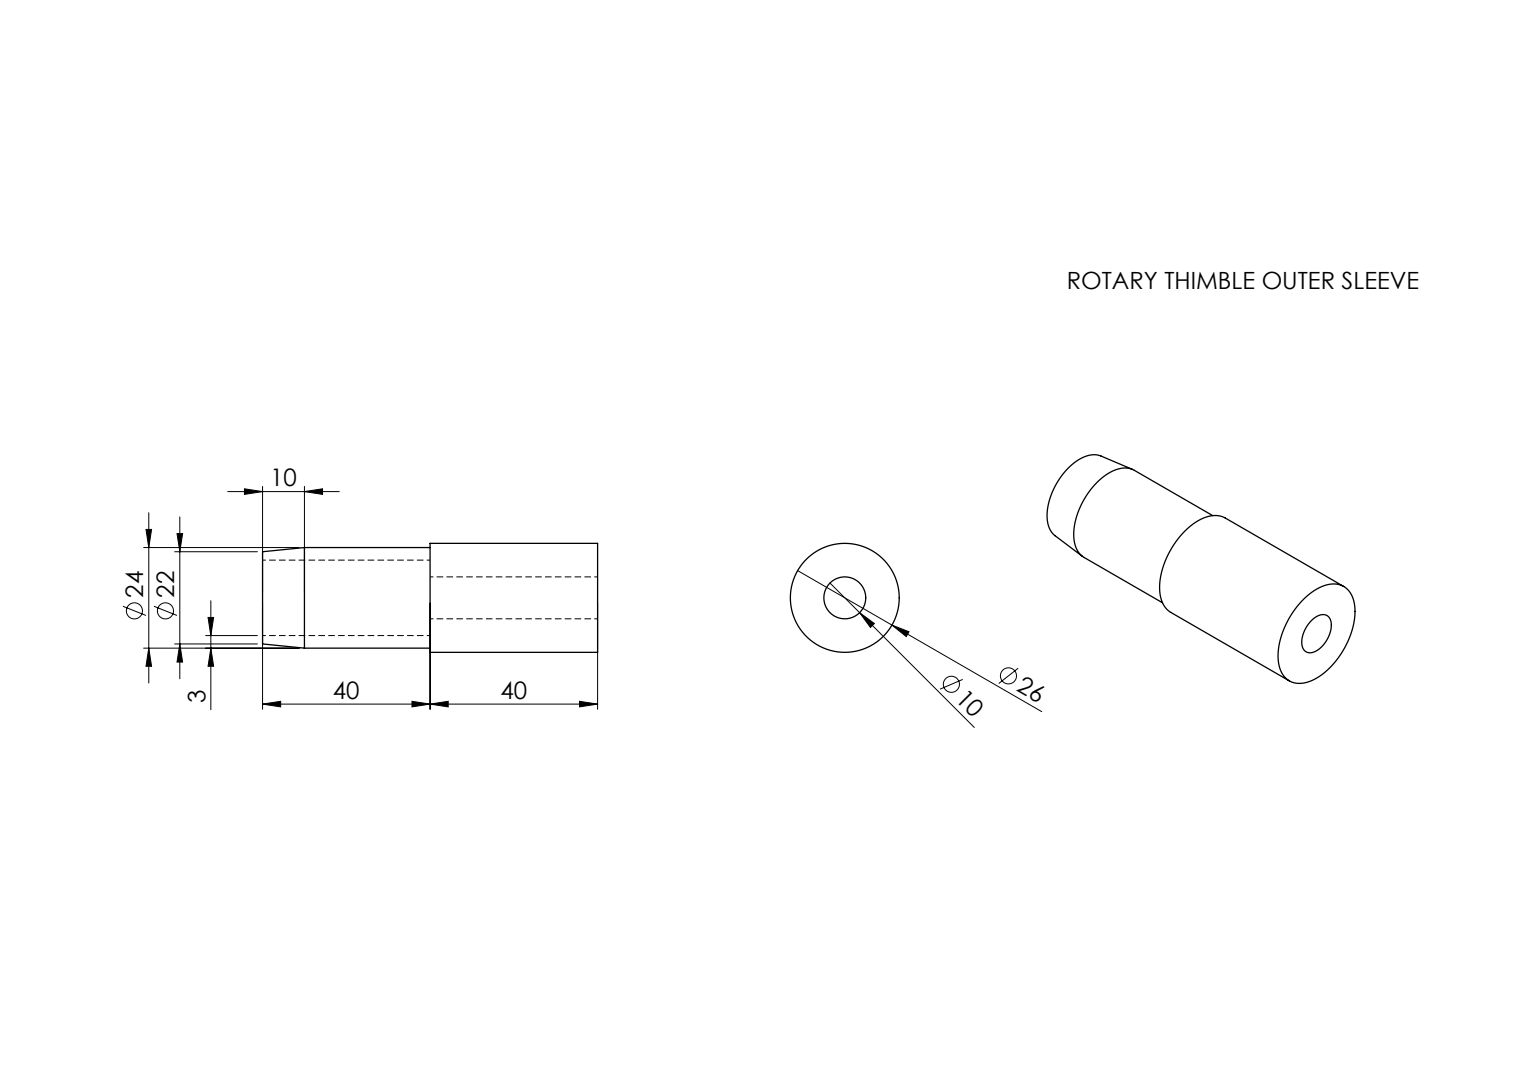
ISO-10303-21;
HEADER;
FILE_DESCRIPTION (('STEP AP214'),
    '1' );
FILE_NAME ('Rotary Thimble Outer Sleeve.step',
    '2026-10-22T12:35:56',
    ( '' ),
    ( '' ),
    'SwSTEP 2.0',
    'SolidWorks 2026',
    '' );
FILE_SCHEMA (( 'AUTOMOTIVE_DESIGN' ));
ENDSEC;

DATA;
#6=CYLINDRICAL_SURFACE ( 'NONE', #446, 5.000000000000000888 ) ;
#10=VECTOR ( 'NONE', #970, 1000.000000000000000 ) ;
#18=STYLED_ITEM ( 'NONE', ( #223 ), #2456 ) ;
#20=LINE ( 'NONE', #2499, #1316 ) ;
#22=EDGE_LOOP ( 'NONE', ( #912, #3109, #1400, #258 ) ) ;
#31=CARTESIAN_POINT ( 'NONE',  ( 100.0000000000000000, -5.826660652933936785E-15, -1.499999999999999556 ) ) ;
#37=SHAPE_REPRESENTATION_RELATIONSHIP ( 'NONE' , 'NONE' ,  #2080, #2456 ) ;
#38=EDGE_LOOP ( 'NONE', ( #1130, #2572 ) ) ;
#65=DIRECTION ( 'NONE',  ( 1.000000000000000000, 0.000000000000000000, 0.000000000000000000 ) ) ;
#83=ORIENTED_EDGE ( 'NONE', *, *, #909, .F. ) ;
#89=CARTESIAN_POINT ( 'NONE',  ( 70.00000000000032685, -6.928842772166554697E-15, 7.500000000000000000 ) ) ;
#92=CARTESIAN_POINT ( 'NONE',  ( 100.0000000000000000, -6.928842772166554697E-15, 7.500000000000000000 ) ) ;
#95=AXIS2_PLACEMENT_3D ( 'NONE', #1120, #2857, #636 ) ;
#104=EDGE_CURVE ( 'NONE', #415, #2077, #2930, .T. ) ;
#105=ORIENTED_EDGE ( 'NONE', *, *, #2070, .F. ) ;
#106=VERTEX_POINT ( 'NONE', #1616 ) ;
#108=VERTEX_POINT ( 'NONE', #3091 ) ;
#114=EDGE_LOOP ( 'NONE', ( #3092, #726, #1252, #1993 ) ) ;
#115=CIRCLE ( 'NONE', #2264, 11.00000000000000355 ) ;
#137=VERTEX_POINT ( 'NONE', #2139 ) ;
#139=DIRECTION ( 'NONE',  ( 0.000000000000000000, 0.000000000000000000, 1.000000000000000000 ) ) ;
#168=PRODUCT_CONTEXT ( 'NONE', #3176, 'mechanical' ) ;
#173=CIRCLE ( 'NONE', #1423, 12.00000000000000000 ) ;
#174=CIRCLE ( 'NONE', #2003, 12.00000000000000000 ) ;
#181=EDGE_LOOP ( 'NONE', ( #2444, #2735 ) ) ;
#183=ORIENTED_EDGE ( 'NONE', *, *, #207, .F. ) ;
#186=CARTESIAN_POINT ( 'NONE',  ( 140.0000000000000000, -6.928842772166554697E-15, 12.50000000000000000 ) ) ;
#192=EDGE_CURVE ( 'NONE', #1084, #211, #1163, .T. ) ;
#205=SURFACE_STYLE_FILL_AREA ( #2455 ) ;
#207=EDGE_CURVE ( 'NONE', #1415, #1866, #1103, .T. ) ;
#209=DIRECTION ( 'NONE',  ( 1.000000000000000000, 0.000000000000000000, 0.000000000000000000 ) ) ;
#211=VERTEX_POINT ( 'NONE', #3209 ) ;
#223=PRESENTATION_STYLE_ASSIGNMENT (( #983 ) ) ;
#230=CIRCLE ( 'NONE', #1844, 13.00000000000000178 ) ;
#236=CARTESIAN_POINT ( 'NONE',  ( 100.0000000000000000, -6.928842772166554697E-15, 19.50000000000000000 ) ) ;
#238=LINE ( 'NONE', #2000, #1057 ) ;
#240=( NAMED_UNIT ( * ) PLANE_ANGLE_UNIT ( ) SI_UNIT ( $, .RADIAN. ) );
#251=DIRECTION ( 'NONE',  ( 0.000000000000000000, 0.000000000000000000, -1.000000000000000000 ) ) ;
#255=LINE ( 'NONE', #1808, #442 ) ;
#258=ORIENTED_EDGE ( 'NONE', *, *, #2595, .F. ) ;
#271=DIRECTION ( 'NONE',  ( -1.000000000000000000, -0.000000000000000000, -0.000000000000000000 ) ) ;
#280=AXIS2_PLACEMENT_3D ( 'NONE', #2473, #2667, #2948 ) ;
#296=ADVANCED_FACE ( 'NONE', ( #1851 ), #6, .F. ) ;
#300=DIRECTION ( 'NONE',  ( 0.000000000000000000, 0.000000000000000000, -1.000000000000000000 ) ) ;
#306=DIRECTION ( 'NONE',  ( -1.000000000000000000, -0.000000000000000000, -0.000000000000000000 ) ) ;
#319=CARTESIAN_POINT ( 'NONE',  ( 100.0000000000000000, -5.826660652933936785E-15, -1.499999999999999556 ) ) ;
#322=DIRECTION ( 'NONE',  ( 0.000000000000000000, 0.000000000000000000, -1.000000000000000000 ) ) ;
#359=VERTEX_POINT ( 'NONE', #740 ) ;
#360=ADVANCED_FACE ( 'NONE', ( #1740 ), #714, .F. ) ;
#364=ORIENTED_EDGE ( 'NONE', *, *, #2262, .F. ) ;
#381=FACE_BOUND ( 'NONE', #577, .T. ) ;
#383=FACE_OUTER_BOUND ( 'NONE', #1369, .T. ) ;
#387=FACE_OUTER_BOUND ( 'NONE', #22, .T. ) ;
#402=CARTESIAN_POINT ( 'NONE',  ( 100.0000000000000000, -6.928842772166554697E-15, 20.50000000000000000 ) ) ;
#405=CYLINDRICAL_SURFACE ( 'NONE', #2026, 12.00000000000000000 ) ;
#413=CARTESIAN_POINT ( 'NONE',  ( 100.0000000000000000, -6.928842772166554697E-15, 7.500000000000000000 ) ) ;
#414=ADVANCED_FACE ( 'NONE', ( #2258 ), #2743, .F. ) ;
#415=VERTEX_POINT ( 'NONE', #482 ) ;
#421=ORIENTED_EDGE ( 'NONE', *, *, #1100, .F. ) ;
#436=EDGE_CURVE ( 'NONE', #1803, #211, #2967, .T. ) ;
#442=VECTOR ( 'NONE', #760, 1000.000000000000000 ) ;
#446=AXIS2_PLACEMENT_3D ( 'NONE', #986, #1989, #749 ) ;
#449=EDGE_LOOP ( 'NONE', ( #2891, #1302, #2981, #2325 ) ) ;
#451=ORIENTED_EDGE ( 'NONE', *, *, #3048, .T. ) ;
#457=DIRECTION ( 'NONE',  ( 0.000000000000000000, 0.000000000000000000, -1.000000000000000000 ) ) ;
#467=LINE ( 'NONE', #3149, #2202 ) ;
#482=CARTESIAN_POINT ( 'NONE',  ( 60.00000000000000000, -6.928842772166554697E-15, 16.50000000000000000 ) ) ;
#493=CIRCLE ( 'NONE', #3140, 12.00000000000000000 ) ;
#494=FACE_OUTER_BOUND ( 'NONE', #181, .T. ) ;
#495=CIRCLE ( 'NONE', #1644, 13.00000000000000178 ) ;
#501=MECHANICAL_DESIGN_GEOMETRIC_PRESENTATION_REPRESENTATION('',(#18),#1537);
#504=PLANE ( 'NONE',  #2021 ) ;
#506=( NAMED_UNIT ( * ) SI_UNIT ( $, .STERADIAN. ) SOLID_ANGLE_UNIT ( ) );
#510=EDGE_CURVE ( 'NONE', #211, #1084, #174, .T. ) ;
#528=CARTESIAN_POINT ( 'NONE',  ( 100.0000000000000000, -5.459266613189731341E-15, -4.500000000000000888 ) ) ;
#536=CYLINDRICAL_SURFACE ( 'NONE', #1581, 13.00000000000000178 ) ;
#543=CIRCLE ( 'NONE', #2666, 9.000000000000000000 ) ;
#546=VERTEX_POINT ( 'NONE', #31 ) ;
#556=CARTESIAN_POINT ( 'NONE',  ( 70.00000000000032685, -6.928842772166554697E-15, 19.50000000000000000 ) ) ;
#563=DIRECTION ( 'NONE',  ( 0.000000000000000000, 0.000000000000000000, -1.000000000000000000 ) ) ;
#570=DIRECTION ( 'NONE',  ( 1.000000000000000000, 0.000000000000000000, 0.000000000000000000 ) ) ;
#577=EDGE_LOOP ( 'NONE', ( #3165, #2114 ) ) ;
#582=DIRECTION ( 'NONE',  ( 0.9950371902099894861, 1.218569110023196515E-17, 0.09950371902099541810 ) ) ;
#590=AXIS2_PLACEMENT_3D ( 'NONE', #2153, #2814, #139 ) ;
#592=AXIS2_PLACEMENT_3D ( 'NONE', #1852, #1310, #2370 ) ;
#619=ORIENTED_EDGE ( 'NONE', *, *, #2326, .F. ) ;
#620=FACE_OUTER_BOUND ( 'NONE', #1333, .T. ) ;
#627=CARTESIAN_POINT ( 'NONE',  ( 140.0000000000000000, -6.316519372592878167E-15, 2.499999999999999556 ) ) ;
#636=DIRECTION ( 'NONE',  ( 0.000000000000000000, 0.000000000000000000, -1.000000000000000000 ) ) ;
#641=DIRECTION ( 'NONE',  ( 1.000000000000000000, 0.000000000000000000, 0.000000000000000000 ) ) ;
#665=EDGE_LOOP ( 'NONE', ( #1180, #1453, #1135, #836 ) ) ;
#692=EDGE_CURVE ( 'NONE', #3085, #1246, #230, .T. ) ;
#703=AXIS2_PLACEMENT_3D ( 'NONE', #1569, #2144, #2570 ) ;
#714=CYLINDRICAL_SURFACE ( 'NONE', #1903, 9.000000000000001776 ) ;
#715=CARTESIAN_POINT ( 'NONE',  ( 140.0000000000000000, -6.316519372592878167E-15, 2.499999999999999556 ) ) ;
#720=SURFACE_SIDE_STYLE ('',( #205 ) ) ;
#726=ORIENTED_EDGE ( 'NONE', *, *, #2442, .F. ) ;
#728=CARTESIAN_POINT ( 'NONE',  ( 100.0000000000000000, -5.459266613189731341E-15, -4.500000000000000888 ) ) ;
#740=CARTESIAN_POINT ( 'NONE',  ( 140.0000000000000000, -6.928842772166554697E-15, 20.50000000000000000 ) ) ;
#749=DIRECTION ( 'NONE',  ( 0.000000000000000000, 0.000000000000000000, 1.000000000000000000 ) ) ;
#760=DIRECTION ( 'NONE',  ( -1.000000000000000000, -0.000000000000000000, -0.000000000000000000 ) ) ;
#788=ADVANCED_FACE ( 'NONE', ( #1081 ), #2634, .T. ) ;
#793=( NAMED_UNIT ( * ) SI_UNIT ( $, .STERADIAN. ) SOLID_ANGLE_UNIT ( ) );
#806=DIRECTION ( 'NONE',  ( 1.000000000000000000, 0.000000000000000000, 0.000000000000000000 ) ) ;
#808=APPLICATION_CONTEXT ( 'automotive_design' ) ;
#811=EDGE_CURVE ( 'NONE', #546, #1226, #543, .T. ) ;
#836=ORIENTED_EDGE ( 'NONE', *, *, #2343, .F. ) ;
#849=CIRCLE ( 'NONE', #2056, 9.000000000000000000 ) ;
#860=DIRECTION ( 'NONE',  ( 1.000000000000000000, 0.000000000000000000, 0.000000000000000000 ) ) ;
#866=EDGE_CURVE ( 'NONE', #106, #137, #2406, .T. ) ;
#904=AXIS2_PLACEMENT_3D ( 'NONE', #2849, #2602, #1075 ) ;
#909=EDGE_CURVE ( 'NONE', #106, #211, #3189, .T. ) ;
#910=COLOUR_RGB ( '',0.8941176470588234615, 0.8941176470588234615, 0.8941176470588234615 ) ;
#912=ORIENTED_EDGE ( 'NONE', *, *, #2361, .F. ) ;
#944=ORIENTED_EDGE ( 'NONE', *, *, #1085, .F. ) ;
#970=DIRECTION ( 'NONE',  ( 0.9950371902099894861, 0.000000000000000000, -0.09950371902099541810 ) ) ;
#983=SURFACE_STYLE_USAGE ( .BOTH. , #720 ) ;
#986=CARTESIAN_POINT ( 'NONE',  ( 140.0000000000000000, -6.928842772166554697E-15, 7.500000000000000000 ) ) ;
#994=ADVANCED_FACE ( 'NONE', ( #1911 ), #1579, .T. ) ;
#1018=ORIENTED_EDGE ( 'NONE', *, *, #866, .F. ) ;
#1028=DIRECTION ( 'NONE',  ( 1.000000000000000000, 0.000000000000000000, 0.000000000000000000 ) ) ;
#1029=CARTESIAN_POINT ( 'NONE',  ( 140.0000000000000000, -6.928842772166554697E-15, 7.500000000000000000 ) ) ;
#1057=VECTOR ( 'NONE', #306, 1000.000000000000000 ) ;
#1064=EDGE_LOOP ( 'NONE', ( #2176, #3018 ) ) ;
#1066=DIRECTION ( 'NONE',  ( 1.000000000000000000, 0.000000000000000000, 0.000000000000000000 ) ) ;
#1075=DIRECTION ( 'NONE',  ( 0.000000000000000000, 0.000000000000000000, -1.000000000000000000 ) ) ;
#1081=FACE_OUTER_BOUND ( 'NONE', #114, .T. ) ;
#1084=VERTEX_POINT ( 'NONE', #556 ) ;
#1085=EDGE_CURVE ( 'NONE', #1226, #415, #20, .T. ) ;
#1089=DIRECTION ( 'NONE',  ( 0.000000000000000000, 0.000000000000000000, -1.000000000000000000 ) ) ;
#1100=EDGE_CURVE ( 'NONE', #2974, #2689, #1442, .T. ) ;
#1103=CIRCLE ( 'NONE', #2209, 5.000000000000000000 ) ;
#1104=EDGE_CURVE ( 'NONE', #108, #1246, #2532, .T. ) ;
#1120=CARTESIAN_POINT ( 'NONE',  ( 140.0000000000000000, -6.928842772166554697E-15, 7.500000000000000000 ) ) ;
#1121=ORIENTED_EDGE ( 'NONE', *, *, #192, .F. ) ;
#1130=ORIENTED_EDGE ( 'NONE', *, *, #104, .T. ) ;
#1131=CARTESIAN_POINT ( 'NONE',  ( 70.00000000000032685, -5.459266613189731341E-15, 19.50000000000000000 ) ) ;
#1135=ORIENTED_EDGE ( 'NONE', *, *, #1085, .T. ) ;
#1137=DIRECTION ( 'NONE',  ( 0.000000000000000000, 0.000000000000000000, -1.000000000000000000 ) ) ;
#1142=FACE_OUTER_BOUND ( 'NONE', #1994, .T. ) ;
#1163=CIRCLE ( 'NONE', #280, 12.00000000000000000 ) ;
#1167=CIRCLE ( 'NONE', #592, 9.000000000000000000 ) ;
#1173=CARTESIAN_POINT ( 'NONE',  ( 70.00000000000032685, -6.928842772166554697E-15, -4.500000000000000888 ) ) ;
#1180=ORIENTED_EDGE ( 'NONE', *, *, #1661, .F. ) ;
#1190=PRODUCT_DEFINITION_CONTEXT ( 'detailed design', #808, 'design' ) ;
#1210=CARTESIAN_POINT ( 'NONE',  ( 100.0000000000000000, -6.928842772166554697E-15, 7.500000000000000000 ) ) ;
#1224=CYLINDRICAL_SURFACE ( 'NONE', #1680, 5.000000000000000888 ) ;
#1226=VERTEX_POINT ( 'NONE', #1354 ) ;
#1242=DIRECTION ( 'NONE',  ( 0.000000000000000000, 0.000000000000000000, 1.000000000000000000 ) ) ;
#1246=VERTEX_POINT ( 'NONE', #3067 ) ;
#1252=ORIENTED_EDGE ( 'NONE', *, *, #2595, .T. ) ;
#1263=ADVANCED_FACE ( 'NONE', ( #387 ), #405, .T. ) ;
#1269=DIRECTION ( 'NONE',  ( 0.000000000000000000, 0.000000000000000000, -1.000000000000000000 ) ) ;
#1275=DIRECTION ( 'NONE',  ( 0.000000000000000000, 0.000000000000000000, -1.000000000000000000 ) ) ;
#1296=( NAMED_UNIT ( * ) PLANE_ANGLE_UNIT ( ) SI_UNIT ( $, .RADIAN. ) );
#1298=DIRECTION ( 'NONE',  ( 1.000000000000000000, 0.000000000000000000, 0.000000000000000000 ) ) ;
#1302=ORIENTED_EDGE ( 'NONE', *, *, #3048, .F. ) ;
#1306=LINE ( 'NONE', #319, #1921 ) ;
#1310=DIRECTION ( 'NONE',  ( 1.000000000000000000, 0.000000000000000000, 0.000000000000000000 ) ) ;
#1316=VECTOR ( 'NONE', #271, 1000.000000000000000 ) ;
#1317=AXIS2_PLACEMENT_3D ( 'NONE', #2581, #2862, #2829 ) ;
#1327=DIRECTION ( 'NONE',  ( -1.000000000000000000, -0.000000000000000000, -0.000000000000000000 ) ) ;
#1333=EDGE_LOOP ( 'NONE', ( #619, #1611, #2598, #83 ) ) ;
#1340=FACE_OUTER_BOUND ( 'NONE', #1064, .T. ) ;
#1354=CARTESIAN_POINT ( 'NONE',  ( 100.0000000000000000, -6.928842772166554697E-15, 16.50000000000000000 ) ) ;
#1366=DIRECTION ( 'NONE',  ( 0.000000000000000000, 0.000000000000000000, -1.000000000000000000 ) ) ;
#1369=EDGE_LOOP ( 'NONE', ( #2626, #1872, #2293, #364 ) ) ;
#1372=DIRECTION ( 'NONE',  ( 0.000000000000000000, 0.000000000000000000, -1.000000000000000000 ) ) ;
#1380=DIRECTION ( 'NONE',  ( 1.000000000000000000, 0.000000000000000000, 0.000000000000000000 ) ) ;
#1391=CARTESIAN_POINT ( 'NONE',  ( 100.0000000000000000, -6.928842772166554697E-15, 7.500000000000000000 ) ) ;
#1400=ORIENTED_EDGE ( 'NONE', *, *, #510, .T. ) ;
#1415=VERTEX_POINT ( 'NONE', #2644 ) ;
#1423=AXIS2_PLACEMENT_3D ( 'NONE', #2115, #65, #3098 ) ;
#1427=( GEOMETRIC_REPRESENTATION_CONTEXT ( 3 ) GLOBAL_UNCERTAINTY_ASSIGNED_CONTEXT ( ( #2498 ) ) GLOBAL_UNIT_ASSIGNED_CONTEXT ( ( #1452, #1664, #3164 ) ) REPRESENTATION_CONTEXT ( 'NONE', 'WORKASPACE' ) );
#1442=CIRCLE ( 'NONE', #3158, 5.000000000000000000 ) ;
#1452=( LENGTH_UNIT ( ) NAMED_UNIT ( * ) SI_UNIT ( .MILLI., .METRE. ) );
#1453=ORIENTED_EDGE ( 'NONE', *, *, #811, .T. ) ;
#1462=FILL_AREA_STYLE_COLOUR ( '', #910 ) ;
#1480=MECHANICAL_DESIGN_GEOMETRIC_PRESENTATION_REPRESENTATION('',(#2108),#1427);
#1486=PLANE ( 'NONE',  #2395 ) ;
#1496=( LENGTH_UNIT ( ) NAMED_UNIT ( * ) SI_UNIT ( .MILLI., .METRE. ) );
#1505=DIRECTION ( 'NONE',  ( -1.000000000000000000, -0.000000000000000000, -0.000000000000000000 ) ) ;
#1524=DIRECTION ( 'NONE',  ( -1.000000000000000000, -0.000000000000000000, -0.000000000000000000 ) ) ;
#1526=DIRECTION ( 'NONE',  ( 0.000000000000000000, 0.000000000000000000, -1.000000000000000000 ) ) ;
#1536=AXIS2_PLACEMENT_3D ( 'NONE', #2756, #1713, #2013 ) ;
#1537=( GEOMETRIC_REPRESENTATION_CONTEXT ( 3 ) GLOBAL_UNCERTAINTY_ASSIGNED_CONTEXT ( ( #2180 ) ) GLOBAL_UNIT_ASSIGNED_CONTEXT ( ( #1496, #1296, #793 ) ) REPRESENTATION_CONTEXT ( 'NONE', 'WORKASPACE' ) );
#1540=PRODUCT_DEFINITION_FORMATION_WITH_SPECIFIED_SOURCE ( 'ANY', '', #2617, .NOT_KNOWN. ) ;
#1565=EDGE_LOOP ( 'NONE', ( #2027, #1018, #3065, #1121 ) ) ;
#1569=CARTESIAN_POINT ( 'NONE',  ( 140.0000000000000000, -6.928842772166554697E-15, 7.500000000000000000 ) ) ;
#1579=CONICAL_SURFACE ( 'NONE', #1635, 12.00000000000000000, 0.09966865249115851311 ) ;
#1581=AXIS2_PLACEMENT_3D ( 'NONE', #2731, #1524, #1242 ) ;
#1586=VECTOR ( 'NONE', #2478, 1000.000000000000000 ) ;
#1590=ADVANCED_FACE ( 'NONE', ( #2046, #3035 ), #504, .T. ) ;
#1603=CARTESIAN_POINT ( 'NONE',  ( 100.0000000000000000, -6.928842772166554697E-15, 7.500000000000000000 ) ) ;
#1610=ORIENTED_EDGE ( 'NONE', *, *, #2361, .T. ) ;
#1611=ORIENTED_EDGE ( 'NONE', *, *, #2298, .T. ) ;
#1616=CARTESIAN_POINT ( 'NONE',  ( 60.00000000000000000, -6.928842772166554697E-15, -3.500000000000003109 ) ) ;
#1635=AXIS2_PLACEMENT_3D ( 'NONE', #1719, #2700, #457 ) ;
#1644=AXIS2_PLACEMENT_3D ( 'NONE', #1902, #860, #2091 ) ;
#1658=ORIENTED_EDGE ( 'NONE', *, *, #1100, .T. ) ;
#1661=EDGE_CURVE ( 'NONE', #546, #2077, #1306, .T. ) ;
#1664=( NAMED_UNIT ( * ) PLANE_ANGLE_UNIT ( ) SI_UNIT ( $, .RADIAN. ) );
#1680=AXIS2_PLACEMENT_3D ( 'NONE', #1962, #2753, #2271 ) ;
#1702=CIRCLE ( 'NONE', #2564, 13.00000000000000178 ) ;
#1713=DIRECTION ( 'NONE',  ( -1.000000000000000000, -0.000000000000000000, -0.000000000000000000 ) ) ;
#1718=ADVANCED_FACE ( 'NONE', ( #381, #1142 ), #1898, .F. ) ;
#1719=CARTESIAN_POINT ( 'NONE',  ( 70.00000000000032685, -6.928842772166554697E-15, 7.500000000000000000 ) ) ;
#1723=FACE_BOUND ( 'NONE', #38, .T. ) ;
#1730=CIRCLE ( 'NONE', #95, 5.000000000000000000 ) ;
#1731=DIRECTION ( 'NONE',  ( -1.000000000000000000, -0.000000000000000000, -0.000000000000000000 ) ) ;
#1736=CARTESIAN_POINT ( 'NONE',  ( 60.00000000000000000, -6.928842772166554697E-15, 7.500000000000000000 ) ) ;
#1740=FACE_OUTER_BOUND ( 'NONE', #665, .T. ) ;
#1746=AXIS2_PLACEMENT_3D ( 'NONE', #92, #2079, #2557 ) ;
#1776=ADVANCED_FACE ( 'NONE', ( #494, #1723 ), #1486, .F. ) ;
#1794=DIRECTION ( 'NONE',  ( 1.000000000000000000, 0.000000000000000000, 0.000000000000000000 ) ) ;
#1803=VERTEX_POINT ( 'NONE', #528 ) ;
#1808=CARTESIAN_POINT ( 'NONE',  ( 140.0000000000000000, -6.928842772166554697E-15, 20.50000000000000000 ) ) ;
#1810=CARTESIAN_POINT ( 'NONE',  ( 140.0000000000000000, -5.336801933274995404E-15, -5.500000000000001776 ) ) ;
#1811=ORIENTED_EDGE ( 'NONE', *, *, #2070, .T. ) ;
#1819=EDGE_LOOP ( 'NONE', ( #451, #2655 ) ) ;
#1826=ADVANCED_FACE ( 'NONE', ( #2240 ), #1224, .F. ) ;
#1837=DIRECTION ( 'NONE',  ( 1.000000000000000000, 0.000000000000000000, 0.000000000000000000 ) ) ;
#1844=AXIS2_PLACEMENT_3D ( 'NONE', #2486, #1298, #3049 ) ;
#1851=FACE_OUTER_BOUND ( 'NONE', #2388, .T. ) ;
#1852=CARTESIAN_POINT ( 'NONE',  ( 60.00000000000000000, -6.928842772166554697E-15, 7.500000000000000000 ) ) ;
#1855=EDGE_LOOP ( 'NONE', ( #2272, #1610 ) ) ;
#1866=VERTEX_POINT ( 'NONE', #2978 ) ;
#1868=DIRECTION ( 'NONE',  ( 0.000000000000000000, 0.000000000000000000, 1.000000000000000000 ) ) ;
#1872=ORIENTED_EDGE ( 'NONE', *, *, #1104, .T. ) ;
#1888=VECTOR ( 'NONE', #2166, 1000.000000000000000 ) ;
#1898=PLANE ( 'NONE',  #2748 ) ;
#1901=ORIENTED_EDGE ( 'NONE', *, *, #2191, .F. ) ;
#1902=CARTESIAN_POINT ( 'NONE',  ( 140.0000000000000000, -6.928842772166554697E-15, 7.500000000000000000 ) ) ;
#1903=AXIS2_PLACEMENT_3D ( 'NONE', #1210, #1505, #2449 ) ;
#1911=FACE_OUTER_BOUND ( 'NONE', #1565, .T. ) ;
#1921=VECTOR ( 'NONE', #2306, 1000.000000000000000 ) ;
#1959=( LENGTH_UNIT ( ) NAMED_UNIT ( * ) SI_UNIT ( .MILLI., .METRE. ) );
#1962=CARTESIAN_POINT ( 'NONE',  ( 140.0000000000000000, -6.928842772166554697E-15, 7.500000000000000000 ) ) ;
#1987=ADVANCED_FACE ( 'NONE', ( #620 ), #2141, .T. ) ;
#1989=DIRECTION ( 'NONE',  ( -1.000000000000000000, -0.000000000000000000, -0.000000000000000000 ) ) ;
#1993=ORIENTED_EDGE ( 'NONE', *, *, #192, .T. ) ;
#1994=EDGE_LOOP ( 'NONE', ( #2692, #2519 ) ) ;
#2000=CARTESIAN_POINT ( 'NONE',  ( 140.0000000000000000, -6.928842772166554697E-15, 12.50000000000000000 ) ) ;
#2003=AXIS2_PLACEMENT_3D ( 'NONE', #89, #2075, #300 ) ;
#2013=DIRECTION ( 'NONE',  ( 0.000000000000000000, 0.000000000000000000, 1.000000000000000000 ) ) ;
#2021=AXIS2_PLACEMENT_3D ( 'NONE', #1029, #806, #251 ) ;
#2026=AXIS2_PLACEMENT_3D ( 'NONE', #1391, #1327, #1868 ) ;
#2027=ORIENTED_EDGE ( 'NONE', *, *, #2298, .F. ) ;
#2046=FACE_OUTER_BOUND ( 'NONE', #1819, .T. ) ;
#2051=AXIS2_PLACEMENT_3D ( 'NONE', #2685, #1731, #2647 ) ;
#2056=AXIS2_PLACEMENT_3D ( 'NONE', #1603, #2368, #1089 ) ;
#2070=EDGE_CURVE ( 'NONE', #2689, #2974, #1730, .T. ) ;
#2075=DIRECTION ( 'NONE',  ( 1.000000000000000000, -0.000000000000000000, -0.000000000000000000 ) ) ;
#2077=VERTEX_POINT ( 'NONE', #2609 ) ;
#2079=DIRECTION ( 'NONE',  ( 1.000000000000000000, 0.000000000000000000, 0.000000000000000000 ) ) ;
#2080=SHAPE_REPRESENTATION ( 'Rotary Thimble Outer Sleeve', ( #2878 ), #2989 ) ;
#2091=DIRECTION ( 'NONE',  ( 0.000000000000000000, 0.000000000000000000, -1.000000000000000000 ) ) ;
#2095=SHAPE_DEFINITION_REPRESENTATION ( #2977, #2080 ) ;
#2108=STYLED_ITEM('',(#3243),#3178);
#2114=ORIENTED_EDGE ( 'NONE', *, *, #207, .T. ) ;
#2115=CARTESIAN_POINT ( 'NONE',  ( 100.0000000000000000, -6.928842772166554697E-15, 7.500000000000000000 ) ) ;
#2127=CYLINDRICAL_SURFACE ( 'NONE', #703, 13.00000000000000178 ) ;
#2139=CARTESIAN_POINT ( 'NONE',  ( 60.00000000000000000, -5.520498953147098126E-15, 18.50000000000000355 ) ) ;
#2141=CONICAL_SURFACE ( 'NONE', #3068, 12.00000000000000000, 0.09966865249115851311 ) ;
#2144=DIRECTION ( 'NONE',  ( -1.000000000000000000, -0.000000000000000000, -0.000000000000000000 ) ) ;
#2153=CARTESIAN_POINT ( 'NONE',  ( 100.0000000000000000, -6.928842772166554697E-15, 7.500000000000000000 ) ) ;
#2156=ORIENTED_EDGE ( 'NONE', *, *, #1661, .T. ) ;
#2166=DIRECTION ( 'NONE',  ( -1.000000000000000000, -0.000000000000000000, -0.000000000000000000 ) ) ;
#2172=ADVANCED_FACE ( 'NONE', ( #2760 ), #536, .T. ) ;
#2176=ORIENTED_EDGE ( 'NONE', *, *, #692, .F. ) ;
#2180=UNCERTAINTY_MEASURE_WITH_UNIT (LENGTH_MEASURE( 1.000000000000000082E-05 ), #1496, 'distance_accuracy_value', 'NONE');
#2191=EDGE_CURVE ( 'NONE', #1866, #1415, #3084, .T. ) ;
#2193=EDGE_CURVE ( 'NONE', #2689, #1866, #238, .T. ) ;
#2195=ORIENTED_EDGE ( 'NONE', *, *, #2193, .F. ) ;
#2202=VECTOR ( 'NONE', #3183, 1000.000000000000000 ) ;
#2204=DIRECTION ( 'NONE',  ( 0.000000000000000000, 0.000000000000000000, -1.000000000000000000 ) ) ;
#2209=AXIS2_PLACEMENT_3D ( 'NONE', #2961, #2715, #2204 ) ;
#2240=FACE_OUTER_BOUND ( 'NONE', #3148, .T. ) ;
#2258=FACE_OUTER_BOUND ( 'NONE', #2754, .T. ) ;
#2262=EDGE_CURVE ( 'NONE', #359, #3085, #255, .T. ) ;
#2263=LINE ( 'NONE', #1131, #2668 ) ;
#2264=AXIS2_PLACEMENT_3D ( 'NONE', #3080, #3112, #1372 ) ;
#2271=DIRECTION ( 'NONE',  ( 0.000000000000000000, 0.000000000000000000, 1.000000000000000000 ) ) ;
#2272=ORIENTED_EDGE ( 'NONE', *, *, #2442, .T. ) ;
#2277=DIRECTION ( 'NONE',  ( 0.000000000000000000, 0.000000000000000000, -1.000000000000000000 ) ) ;
#2291=CARTESIAN_POINT ( 'NONE',  ( 100.0000000000000000, -6.928842772166554697E-15, 7.500000000000000000 ) ) ;
#2293=ORIENTED_EDGE ( 'NONE', *, *, #2906, .T. ) ;
#2298=EDGE_CURVE ( 'NONE', #137, #1084, #2263, .T. ) ;
#2306=DIRECTION ( 'NONE',  ( -1.000000000000000000, -0.000000000000000000, -0.000000000000000000 ) ) ;
#2321=CARTESIAN_POINT ( 'NONE',  ( 100.0000000000000000, -6.928842772166554697E-15, 7.500000000000000000 ) ) ;
#2325=ORIENTED_EDGE ( 'NONE', *, *, #692, .T. ) ;
#2326=EDGE_CURVE ( 'NONE', #137, #106, #115, .T. ) ;
#2336=PLANE ( 'NONE',  #1746 ) ;
#2343=EDGE_CURVE ( 'NONE', #2077, #415, #1167, .T. ) ;
#2361=EDGE_CURVE ( 'NONE', #1803, #2769, #493, .T. ) ;
#2368=DIRECTION ( 'NONE',  ( 1.000000000000000000, 0.000000000000000000, 0.000000000000000000 ) ) ;
#2370=DIRECTION ( 'NONE',  ( 0.000000000000000000, 0.000000000000000000, -1.000000000000000000 ) ) ;
#2388=EDGE_LOOP ( 'NONE', ( #2855, #1658, #2980, #183 ) ) ;
#2392=ADVANCED_FACE ( 'NONE', ( #2869, #1340 ), #2336, .F. ) ;
#2395=AXIS2_PLACEMENT_3D ( 'NONE', #1736, #209, #1269 ) ;
#2406=CIRCLE ( 'NONE', #2051, 11.00000000000000355 ) ;
#2413=ORIENTED_EDGE ( 'NONE', *, *, #3060, .T. ) ;
#2442=EDGE_CURVE ( 'NONE', #2769, #1803, #173, .T. ) ;
#2444=ORIENTED_EDGE ( 'NONE', *, *, #866, .T. ) ;
#2449=DIRECTION ( 'NONE',  ( 0.000000000000000000, 0.000000000000000000, 1.000000000000000000 ) ) ;
#2455=FILL_AREA_STYLE ('',( #1462 ) ) ;
#2456=ADVANCED_BREP_SHAPE_REPRESENTATION ( '', ( #3178, #2878 ), #2989 ) ;
#2473=CARTESIAN_POINT ( 'NONE',  ( 70.00000000000032685, -6.928842772166554697E-15, 7.500000000000000000 ) ) ;
#2476=ORIENTED_EDGE ( 'NONE', *, *, #2714, .T. ) ;
#2478=DIRECTION ( 'NONE',  ( -1.000000000000000000, -0.000000000000000000, -0.000000000000000000 ) ) ;
#2482=CARTESIAN_POINT ( 'NONE',  ( 100.0000000000000000, -6.928842772166554697E-15, 7.500000000000000000 ) ) ;
#2486=CARTESIAN_POINT ( 'NONE',  ( 100.0000000000000000, -6.928842772166554697E-15, 7.500000000000000000 ) ) ;
#2498=UNCERTAINTY_MEASURE_WITH_UNIT (LENGTH_MEASURE( 1.000000000000000082E-05 ), #1452, 'distance_accuracy_value', 'NONE');
#2499=CARTESIAN_POINT ( 'NONE',  ( 100.0000000000000000, -6.928842772166554697E-15, 16.50000000000000000 ) ) ;
#2519=ORIENTED_EDGE ( 'NONE', *, *, #811, .F. ) ;
#2532=LINE ( 'NONE', #1810, #2844 ) ;
#2557=DIRECTION ( 'NONE',  ( 0.000000000000000000, 0.000000000000000000, -1.000000000000000000 ) ) ;
#2564=AXIS2_PLACEMENT_3D ( 'NONE', #2291, #1028, #1275 ) ;
#2570=DIRECTION ( 'NONE',  ( 0.000000000000000000, 0.000000000000000000, 1.000000000000000000 ) ) ;
#2572=ORIENTED_EDGE ( 'NONE', *, *, #2343, .T. ) ;
#2581=CARTESIAN_POINT ( 'NONE',  ( 60.00000000000000000, -6.928842772166554697E-15, 7.500000000000000000 ) ) ;
#2595=EDGE_CURVE ( 'NONE', #2769, #1084, #467, .T. ) ;
#2598=ORIENTED_EDGE ( 'NONE', *, *, #510, .F. ) ;
#2602=DIRECTION ( 'NONE',  ( 1.000000000000000000, 0.000000000000000000, 0.000000000000000000 ) ) ;
#2609=CARTESIAN_POINT ( 'NONE',  ( 60.00000000000000000, -5.826660652933936785E-15, -1.499999999999999556 ) ) ;
#2617=PRODUCT ( 'Rotary Thimble Outer Sleeve', 'Rotary Thimble Outer Sleeve', '', ( #168 ) ) ;
#2626=ORIENTED_EDGE ( 'NONE', *, *, #3019, .F. ) ;
#2634=CYLINDRICAL_SURFACE ( 'NONE', #590, 12.00000000000000000 ) ;
#2644=CARTESIAN_POINT ( 'NONE',  ( 100.0000000000000000, -6.316519372592878167E-15, 2.499999999999999556 ) ) ;
#2647=DIRECTION ( 'NONE',  ( 0.000000000000000000, 0.000000000000000000, -1.000000000000000000 ) ) ;
#2655=ORIENTED_EDGE ( 'NONE', *, *, #3019, .T. ) ;
#2658=UNCERTAINTY_MEASURE_WITH_UNIT (LENGTH_MEASURE( 1.000000000000000082E-05 ), #1959, 'distance_accuracy_value', 'NONE');
#2659=LINE ( 'NONE', #715, #1888 ) ;
#2666=AXIS2_PLACEMENT_3D ( 'NONE', #3086, #1380, #1137 ) ;
#2667=DIRECTION ( 'NONE',  ( 1.000000000000000000, -0.000000000000000000, -0.000000000000000000 ) ) ;
#2668=VECTOR ( 'NONE', #582, 1000.000000000000000 ) ;
#2685=CARTESIAN_POINT ( 'NONE',  ( 60.00000000000000000, -6.928842772166554697E-15, 7.500000000000000000 ) ) ;
#2689=VERTEX_POINT ( 'NONE', #186 ) ;
#2692=ORIENTED_EDGE ( 'NONE', *, *, #3060, .F. ) ;
#2700=DIRECTION ( 'NONE',  ( 1.000000000000000000, -0.000000000000000000, -0.000000000000000000 ) ) ;
#2714=EDGE_CURVE ( 'NONE', #2974, #1415, #2659, .T. ) ;
#2715=DIRECTION ( 'NONE',  ( 1.000000000000000000, 0.000000000000000000, 0.000000000000000000 ) ) ;
#2719=ORIENTED_EDGE ( 'NONE', *, *, #104, .F. ) ;
#2731=CARTESIAN_POINT ( 'NONE',  ( 140.0000000000000000, -6.928842772166554697E-15, 7.500000000000000000 ) ) ;
#2735=ORIENTED_EDGE ( 'NONE', *, *, #2326, .T. ) ;
#2743=CYLINDRICAL_SURFACE ( 'NONE', #1536, 9.000000000000001776 ) ;
#2748=AXIS2_PLACEMENT_3D ( 'NONE', #413, #641, #1366 ) ;
#2753=DIRECTION ( 'NONE',  ( -1.000000000000000000, -0.000000000000000000, -0.000000000000000000 ) ) ;
#2754=EDGE_LOOP ( 'NONE', ( #2413, #2156, #2719, #944 ) ) ;
#2756=CARTESIAN_POINT ( 'NONE',  ( 100.0000000000000000, -6.928842772166554697E-15, 7.500000000000000000 ) ) ;
#2760=FACE_OUTER_BOUND ( 'NONE', #449, .T. ) ;
#2769=VERTEX_POINT ( 'NONE', #236 ) ;
#2793=DIRECTION ( 'NONE',  ( -1.000000000000000000, -0.000000000000000000, -0.000000000000000000 ) ) ;
#2799=DIRECTION ( 'NONE',  ( 0.000000000000000000, 0.000000000000000000, 1.000000000000000000 ) ) ;
#2814=DIRECTION ( 'NONE',  ( -1.000000000000000000, -0.000000000000000000, -0.000000000000000000 ) ) ;
#2829=DIRECTION ( 'NONE',  ( 0.000000000000000000, 0.000000000000000000, -1.000000000000000000 ) ) ;
#2844=VECTOR ( 'NONE', #2793, 1000.000000000000000 ) ;
#2849=CARTESIAN_POINT ( 'NONE',  ( 140.0000000000000000, -6.928842772166554697E-15, 7.500000000000000000 ) ) ;
#2854=PRODUCT_DEFINITION ( 'UNKNOWN', '', #1540, #1190 ) ;
#2855=ORIENTED_EDGE ( 'NONE', *, *, #2714, .F. ) ;
#2857=DIRECTION ( 'NONE',  ( 1.000000000000000000, 0.000000000000000000, 0.000000000000000000 ) ) ;
#2862=DIRECTION ( 'NONE',  ( 1.000000000000000000, 0.000000000000000000, 0.000000000000000000 ) ) ;
#2869=FACE_BOUND ( 'NONE', #1855, .T. ) ;
#2873=CARTESIAN_POINT ( 'NONE',  ( 70.00000000000032685, -6.928842772166554697E-15, 7.500000000000000000 ) ) ;
#2878=AXIS2_PLACEMENT_3D ( 'NONE', #3071, #2799, #1837 ) ;
#2891=ORIENTED_EDGE ( 'NONE', *, *, #1104, .F. ) ;
#2906=EDGE_CURVE ( 'NONE', #1246, #3085, #1702, .T. ) ;
#2930=CIRCLE ( 'NONE', #1317, 9.000000000000000000 ) ;
#2932=AXIS2_PLACEMENT_3D ( 'NONE', #2482, #570, #2277 ) ;
#2948=DIRECTION ( 'NONE',  ( 0.000000000000000000, 0.000000000000000000, -1.000000000000000000 ) ) ;
#2959=ADVANCED_FACE ( 'NONE', ( #383 ), #2127, .T. ) ;
#2961=CARTESIAN_POINT ( 'NONE',  ( 100.0000000000000000, -6.928842772166554697E-15, 7.500000000000000000 ) ) ;
#2967=LINE ( 'NONE', #728, #1586 ) ;
#2974=VERTEX_POINT ( 'NONE', #627 ) ;
#2977=PRODUCT_DEFINITION_SHAPE ( 'NONE', 'NONE',  #2854 ) ;
#2978=CARTESIAN_POINT ( 'NONE',  ( 100.0000000000000000, -6.928842772166554697E-15, 12.50000000000000000 ) ) ;
#2980=ORIENTED_EDGE ( 'NONE', *, *, #2193, .T. ) ;
#2981=ORIENTED_EDGE ( 'NONE', *, *, #2262, .T. ) ;
#2983=CIRCLE ( 'NONE', #904, 13.00000000000000178 ) ;
#2989=( GEOMETRIC_REPRESENTATION_CONTEXT ( 3 ) GLOBAL_UNCERTAINTY_ASSIGNED_CONTEXT ( ( #2658 ) ) GLOBAL_UNIT_ASSIGNED_CONTEXT ( ( #1959, #240, #506 ) ) REPRESENTATION_CONTEXT ( 'NONE', 'WORKASPACE' ) );
#3008=EDGE_LOOP ( 'NONE', ( #105, #421 ) ) ;
#3018=ORIENTED_EDGE ( 'NONE', *, *, #2906, .F. ) ;
#3019=EDGE_CURVE ( 'NONE', #108, #359, #495, .T. ) ;
#3021=CARTESIAN_POINT ( 'NONE',  ( 140.0000000000000000, -6.928842772166554697E-15, 7.500000000000000000 ) ) ;
#3035=FACE_BOUND ( 'NONE', #3008, .T. ) ;
#3036=CLOSED_SHELL ( 'NONE', ( #1826, #2959, #1987, #414, #1263, #1776, #788, #360, #994, #1718, #1590, #2392, #2172, #296 ) ) ;
#3048=EDGE_CURVE ( 'NONE', #359, #108, #2983, .T. ) ;
#3049=DIRECTION ( 'NONE',  ( 0.000000000000000000, 0.000000000000000000, -1.000000000000000000 ) ) ;
#3060=EDGE_CURVE ( 'NONE', #1226, #546, #849, .T. ) ;
#3065=ORIENTED_EDGE ( 'NONE', *, *, #909, .T. ) ;
#3067=CARTESIAN_POINT ( 'NONE',  ( 100.0000000000000000, -5.336801933274995404E-15, -5.500000000000001776 ) ) ;
#3068=AXIS2_PLACEMENT_3D ( 'NONE', #2873, #3102, #563 ) ;
#3071=CARTESIAN_POINT ( 'NONE',  ( 0.000000000000000000, 0.000000000000000000, 0.000000000000000000 ) ) ;
#3080=CARTESIAN_POINT ( 'NONE',  ( 60.00000000000000000, -6.928842772166554697E-15, 7.500000000000000000 ) ) ;
#3084=CIRCLE ( 'NONE', #2932, 5.000000000000000000 ) ;
#3085=VERTEX_POINT ( 'NONE', #402 ) ;
#3086=CARTESIAN_POINT ( 'NONE',  ( 100.0000000000000000, -6.928842772166554697E-15, 7.500000000000000000 ) ) ;
#3091=CARTESIAN_POINT ( 'NONE',  ( 140.0000000000000000, -5.336801933274995404E-15, -5.500000000000001776 ) ) ;
#3092=ORIENTED_EDGE ( 'NONE', *, *, #436, .F. ) ;
#3098=DIRECTION ( 'NONE',  ( 0.000000000000000000, 0.000000000000000000, -1.000000000000000000 ) ) ;
#3102=DIRECTION ( 'NONE',  ( 1.000000000000000000, -0.000000000000000000, -0.000000000000000000 ) ) ;
#3109=ORIENTED_EDGE ( 'NONE', *, *, #436, .T. ) ;
#3112=DIRECTION ( 'NONE',  ( -1.000000000000000000, -0.000000000000000000, -0.000000000000000000 ) ) ;
#3140=AXIS2_PLACEMENT_3D ( 'NONE', #2321, #1066, #322 ) ;
#3148=EDGE_LOOP ( 'NONE', ( #1811, #2476, #1901, #2195 ) ) ;
#3149=CARTESIAN_POINT ( 'NONE',  ( 100.0000000000000000, -6.928842772166554697E-15, 19.50000000000000000 ) ) ;
#3158=AXIS2_PLACEMENT_3D ( 'NONE', #3021, #1794, #1526 ) ;
#3164=( NAMED_UNIT ( * ) SI_UNIT ( $, .STERADIAN. ) SOLID_ANGLE_UNIT ( ) );
#3165=ORIENTED_EDGE ( 'NONE', *, *, #2191, .T. ) ;
#3176=APPLICATION_CONTEXT ( 'automotive_design' ) ;
#3178=MANIFOLD_SOLID_BREP ( 'Boss-Extrude1', #3036 ) ;
#3183=DIRECTION ( 'NONE',  ( -1.000000000000000000, -0.000000000000000000, -0.000000000000000000 ) ) ;
#3189=LINE ( 'NONE', #1173, #10 ) ;
#3209=CARTESIAN_POINT ( 'NONE',  ( 70.00000000000032685, -5.459266613189731341E-15, -4.500000000000000888 ) ) ;
#3237=COLOUR_RGB('Light Blue',0.38,0.62,0.78);
#3238=FILL_AREA_STYLE_COLOUR('',#3237);
#3239=FILL_AREA_STYLE('',(#3238));
#3240=SURFACE_STYLE_FILL_AREA(#3239);
#3241=SURFACE_SIDE_STYLE('',(#3240));
#3242=SURFACE_STYLE_USAGE(.BOTH.,#3241);
#3243=PRESENTATION_STYLE_ASSIGNMENT((#3242));
ENDSEC;
END-ISO-10303-21;
